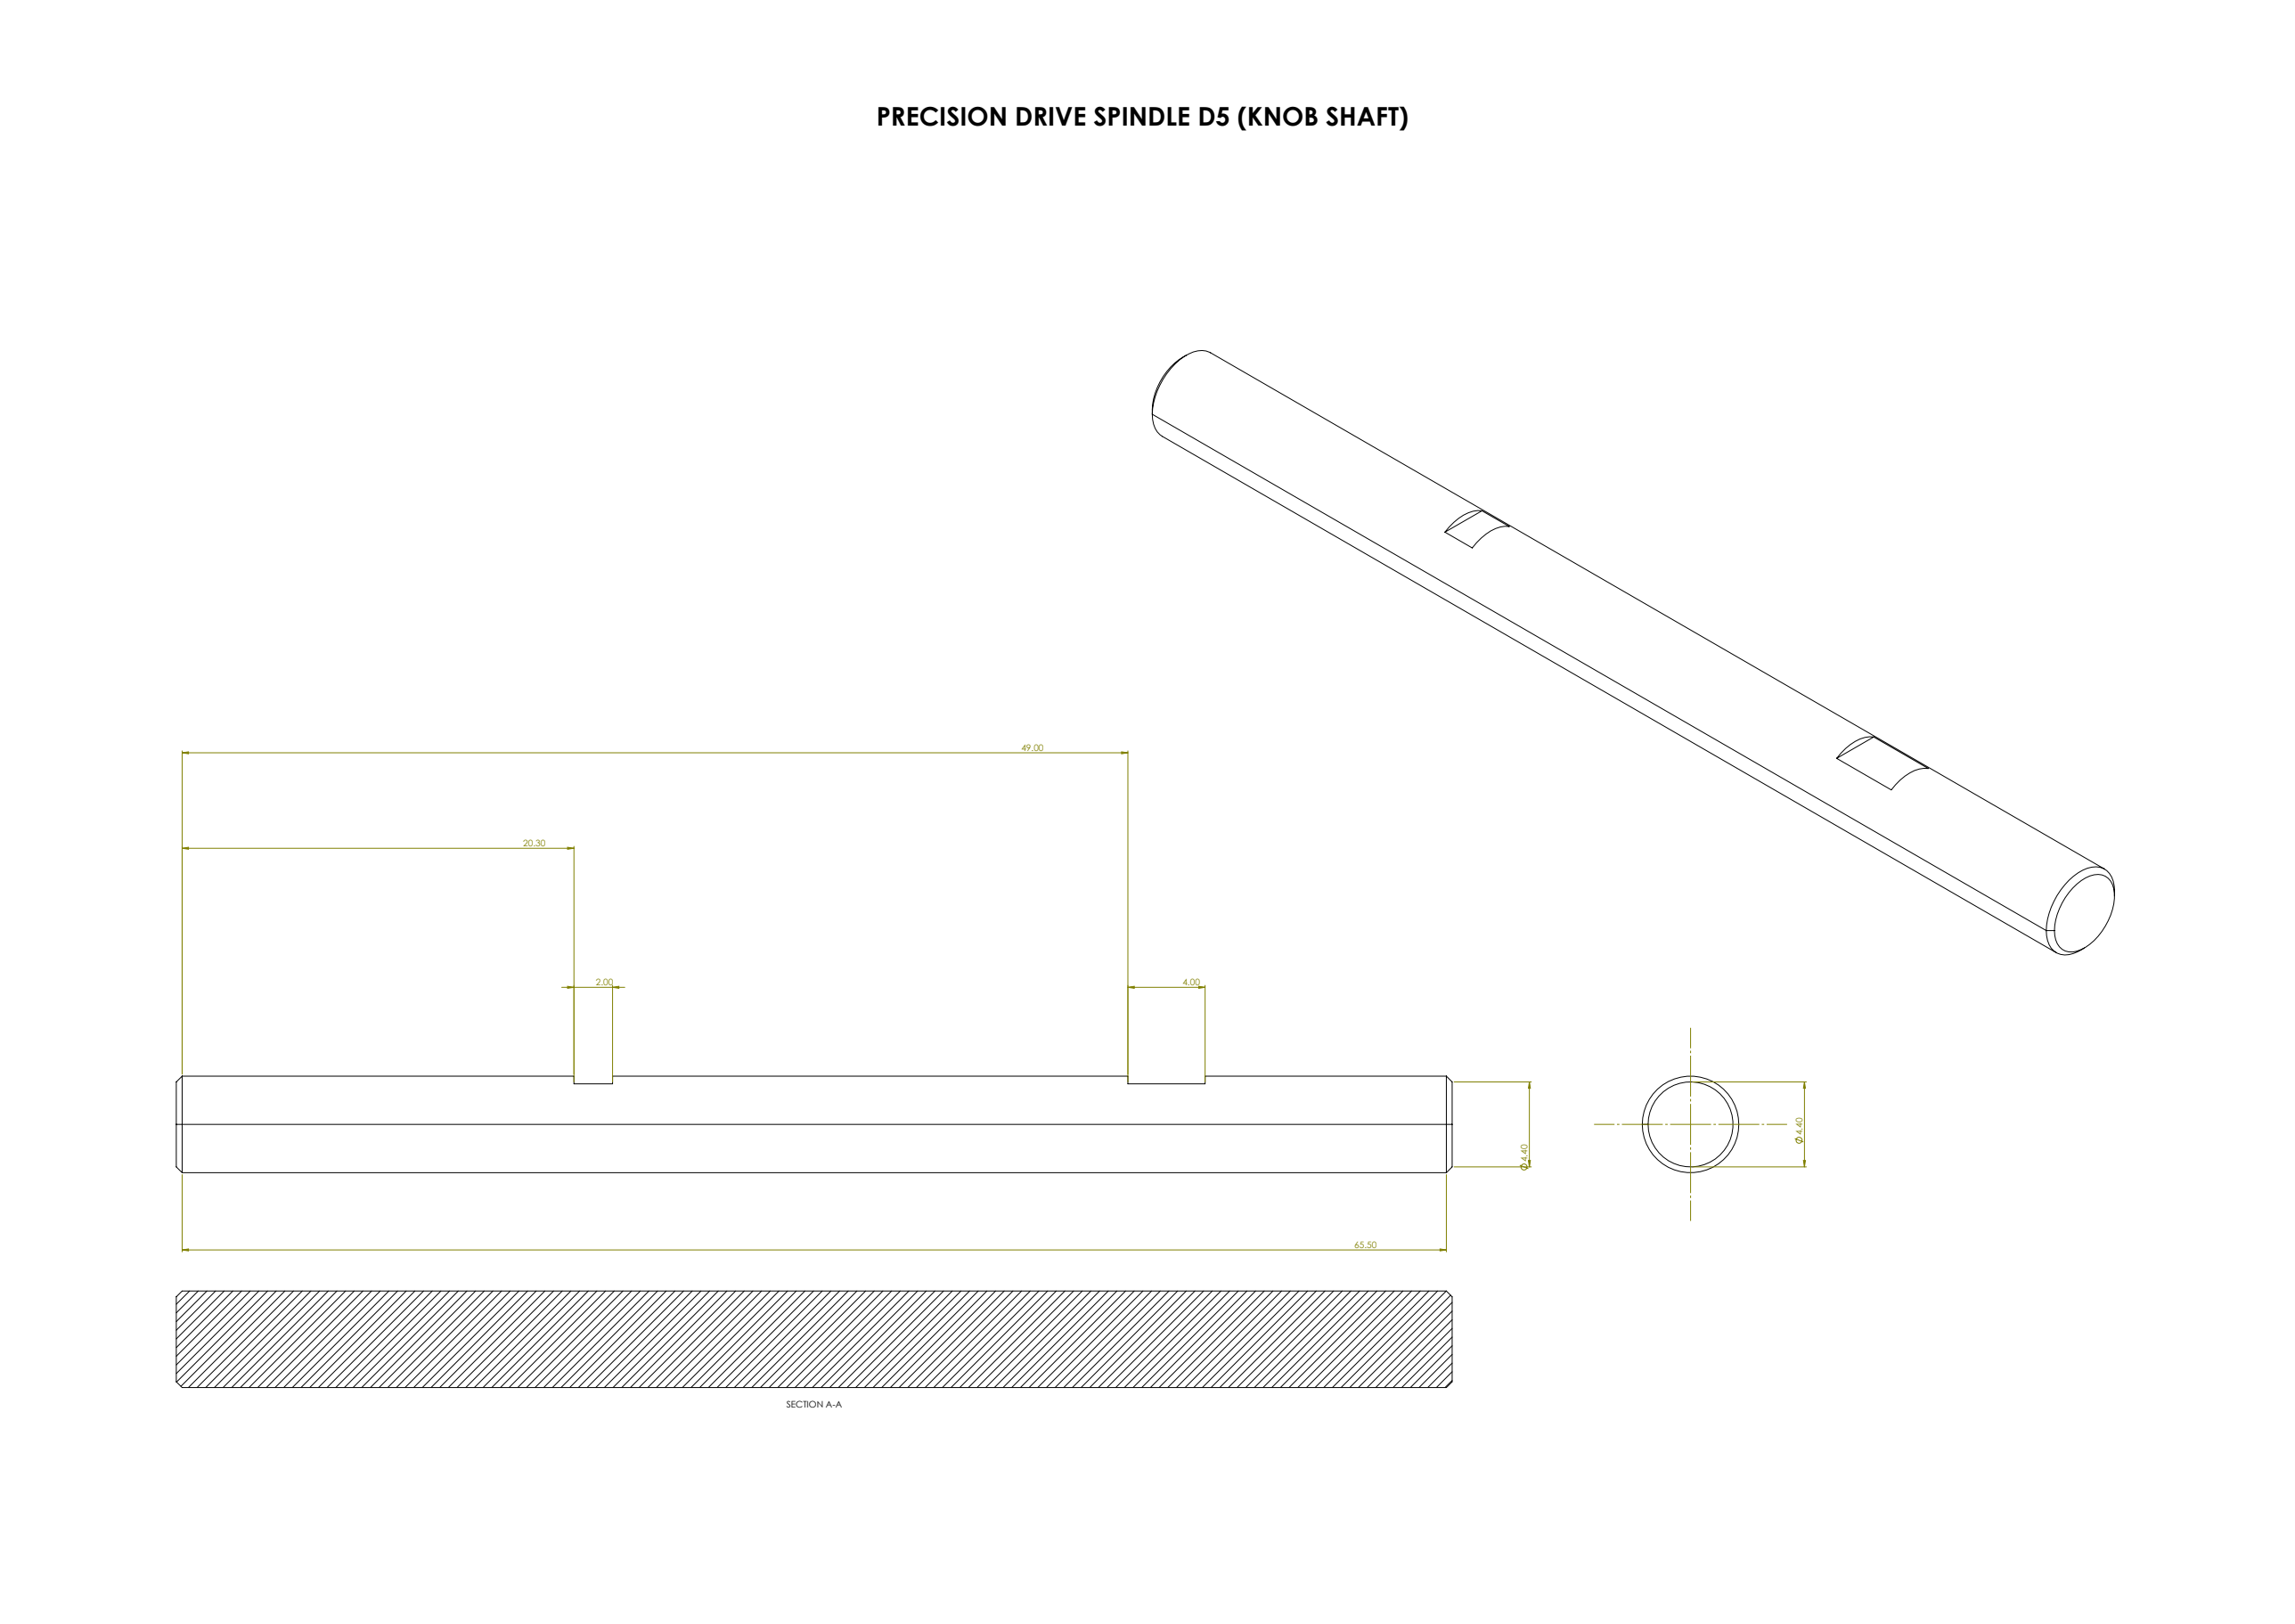
ISO-10303-21;
HEADER;
/* Generated by software containing ST-Developer
 * from STEP Tools, Inc. (www.steptools.com) 
 */

FILE_DESCRIPTION(
/* description */ (''),
/* implementation_level */ '2;1');

FILE_NAME(
/* name */ 'Precision Drive Spindle D5 (knob shaft).step',
/* time_stamp */ '2026-10-05T09:57:53+05:00',
/* author */ (''),
/* organization */ (''),
/* preprocessor_version */ 'ST-DEVELOPER v20.2',
/* originating_system */ 'Autodesk Translation Framework v15.15.0.0',
/* authorisation */ '');

FILE_SCHEMA (('AUTOMOTIVE_DESIGN { 1 0 10303 214 3 1 1 }'));
ENDSEC;

DATA;
#10=MECHANICAL_DESIGN_GEOMETRIC_PRESENTATION_REPRESENTATION('',(#554),#113984);
#518=SHAPE_REPRESENTATION_RELATIONSHIP('SRR','None',#114055,#536);
#536=ADVANCED_BREP_SHAPE_REPRESENTATION('',(#572),#113969);
#554=STYLED_ITEM('',(#114310),#572);
#572=MANIFOLD_SOLID_BREP('Precision Drive Spindle D5 (knob shaft)',#60395);
#635=CYLINDRICAL_SURFACE('',#61984,2.5);
#911=CONICAL_SURFACE('',#61982,2.34999999999999,0.785398163397437);
#912=CONICAL_SURFACE('',#61986,2.34999999999999,0.785398163397448);
#1055=CIRCLE('',#61971,2.5);
#1056=CIRCLE('',#61973,2.5);
#1057=CIRCLE('',#61976,2.5);
#1058=CIRCLE('',#61978,2.5);
#1059=CIRCLE('',#61981,2.20000000000001);
#1060=CIRCLE('',#61983,2.5);
#1061=CIRCLE('',#61985,2.5);
#1062=CIRCLE('',#61987,2.20000000000001);
#1825=FACE_BOUND('',#9526,.T.);
#1826=FACE_BOUND('',#9527,.T.);
#3035=PLANE('',#61970);
#3036=PLANE('',#61972);
#3037=PLANE('',#61974);
#3038=PLANE('',#61975);
#3039=PLANE('',#61977);
#3040=PLANE('',#61979);
#3041=PLANE('',#61980);
#3042=PLANE('',#61988);
#5967=FACE_OUTER_BOUND('',#9517,.T.);
#5968=FACE_OUTER_BOUND('',#9518,.T.);
#5969=FACE_OUTER_BOUND('',#9519,.T.);
#5970=FACE_OUTER_BOUND('',#9520,.T.);
#5971=FACE_OUTER_BOUND('',#9521,.T.);
#5972=FACE_OUTER_BOUND('',#9522,.T.);
#5973=FACE_OUTER_BOUND('',#9523,.T.);
#5974=FACE_OUTER_BOUND('',#9524,.T.);
#5975=FACE_OUTER_BOUND('',#9525,.T.);
#5976=FACE_OUTER_BOUND('',#9528,.T.);
#5977=FACE_OUTER_BOUND('',#9529,.T.);
#9517=EDGE_LOOP('',(#48949,#48950));
#9518=EDGE_LOOP('',(#48951,#48952));
#9519=EDGE_LOOP('',(#48953,#48954,#48955,#48956));
#9520=EDGE_LOOP('',(#48957,#48958));
#9521=EDGE_LOOP('',(#48959,#48960));
#9522=EDGE_LOOP('',(#48961,#48962,#48963,#48964));
#9523=EDGE_LOOP('',(#48965));
#9524=EDGE_LOOP('',(#48966,#48967,#48968,#48969));
#9525=EDGE_LOOP('',(#48970,#48971,#48972,#48973));
#9526=EDGE_LOOP('',(#48974,#48975,#48976,#48977));
#9527=EDGE_LOOP('',(#48978,#48979,#48980,#48981));
#9528=EDGE_LOOP('',(#48982,#48983,#48984,#48985));
#9529=EDGE_LOOP('',(#48986));
#14318=LINE('',#92618,#20352);
#14319=LINE('',#92623,#20353);
#14320=LINE('',#92625,#20354);
#14321=LINE('',#92626,#20355);
#14322=LINE('',#92631,#20356);
#14323=LINE('',#92636,#20357);
#14324=LINE('',#92638,#20358);
#14325=LINE('',#92639,#20359);
#14326=LINE('',#92646,#20360);
#14327=LINE('',#92650,#20361);
#14328=LINE('',#92654,#20362);
#20352=VECTOR('',#69944,10.);
#20353=VECTOR('',#69949,10.);
#20354=VECTOR('',#69952,10.);
#20355=VECTOR('',#69953,10.);
#20356=VECTOR('',#69958,10.);
#20357=VECTOR('',#69963,10.);
#20358=VECTOR('',#69966,10.);
#20359=VECTOR('',#69967,10.);
#20360=VECTOR('',#69976,2.34999999999999);
#20361=VECTOR('',#69981,2.5);
#20362=VECTOR('',#69986,2.34999999999999);
#27899=VERTEX_POINT('',#92615);
#27900=VERTEX_POINT('',#92616);
#27901=VERTEX_POINT('',#92620);
#27902=VERTEX_POINT('',#92621);
#27903=VERTEX_POINT('',#92628);
#27904=VERTEX_POINT('',#92629);
#27905=VERTEX_POINT('',#92633);
#27906=VERTEX_POINT('',#92634);
#27907=VERTEX_POINT('',#92641);
#27908=VERTEX_POINT('',#92644);
#27909=VERTEX_POINT('',#92648);
#27910=VERTEX_POINT('',#92652);
#35307=EDGE_CURVE('',#27899,#27900,#1055,.T.);
#35308=EDGE_CURVE('',#27899,#27900,#14318,.T.);
#35309=EDGE_CURVE('',#27901,#27902,#1056,.T.);
#35310=EDGE_CURVE('',#27901,#27902,#14319,.T.);
#35311=EDGE_CURVE('',#27902,#27899,#14320,.T.);
#35312=EDGE_CURVE('',#27900,#27901,#14321,.T.);
#35313=EDGE_CURVE('',#27903,#27904,#1057,.T.);
#35314=EDGE_CURVE('',#27903,#27904,#14322,.T.);
#35315=EDGE_CURVE('',#27905,#27906,#1058,.T.);
#35316=EDGE_CURVE('',#27905,#27906,#14323,.T.);
#35317=EDGE_CURVE('',#27906,#27903,#14324,.T.);
#35318=EDGE_CURVE('',#27904,#27905,#14325,.T.);
#35319=EDGE_CURVE('',#27907,#27907,#1059,.T.);
#35320=EDGE_CURVE('',#27908,#27908,#1060,.T.);
#35321=EDGE_CURVE('',#27908,#27907,#14326,.T.);
#35322=EDGE_CURVE('',#27909,#27909,#1061,.T.);
#35323=EDGE_CURVE('',#27909,#27908,#14327,.T.);
#35324=EDGE_CURVE('',#27910,#27910,#1062,.T.);
#35325=EDGE_CURVE('',#27910,#27909,#14328,.T.);
#48949=ORIENTED_EDGE('',*,*,#35307,.F.);
#48950=ORIENTED_EDGE('',*,*,#35308,.T.);
#48951=ORIENTED_EDGE('',*,*,#35309,.F.);
#48952=ORIENTED_EDGE('',*,*,#35310,.T.);
#48953=ORIENTED_EDGE('',*,*,#35311,.F.);
#48954=ORIENTED_EDGE('',*,*,#35310,.F.);
#48955=ORIENTED_EDGE('',*,*,#35312,.F.);
#48956=ORIENTED_EDGE('',*,*,#35308,.F.);
#48957=ORIENTED_EDGE('',*,*,#35313,.F.);
#48958=ORIENTED_EDGE('',*,*,#35314,.T.);
#48959=ORIENTED_EDGE('',*,*,#35315,.F.);
#48960=ORIENTED_EDGE('',*,*,#35316,.T.);
#48961=ORIENTED_EDGE('',*,*,#35317,.F.);
#48962=ORIENTED_EDGE('',*,*,#35316,.F.);
#48963=ORIENTED_EDGE('',*,*,#35318,.F.);
#48964=ORIENTED_EDGE('',*,*,#35314,.F.);
#48965=ORIENTED_EDGE('',*,*,#35319,.F.);
#48966=ORIENTED_EDGE('',*,*,#35320,.F.);
#48967=ORIENTED_EDGE('',*,*,#35321,.T.);
#48968=ORIENTED_EDGE('',*,*,#35319,.T.);
#48969=ORIENTED_EDGE('',*,*,#35321,.F.);
#48970=ORIENTED_EDGE('',*,*,#35322,.F.);
#48971=ORIENTED_EDGE('',*,*,#35323,.T.);
#48972=ORIENTED_EDGE('',*,*,#35320,.T.);
#48973=ORIENTED_EDGE('',*,*,#35323,.F.);
#48974=ORIENTED_EDGE('',*,*,#35309,.T.);
#48975=ORIENTED_EDGE('',*,*,#35311,.T.);
#48976=ORIENTED_EDGE('',*,*,#35307,.T.);
#48977=ORIENTED_EDGE('',*,*,#35312,.T.);
#48978=ORIENTED_EDGE('',*,*,#35315,.T.);
#48979=ORIENTED_EDGE('',*,*,#35317,.T.);
#48980=ORIENTED_EDGE('',*,*,#35313,.T.);
#48981=ORIENTED_EDGE('',*,*,#35318,.T.);
#48982=ORIENTED_EDGE('',*,*,#35324,.F.);
#48983=ORIENTED_EDGE('',*,*,#35325,.T.);
#48984=ORIENTED_EDGE('',*,*,#35322,.T.);
#48985=ORIENTED_EDGE('',*,*,#35325,.F.);
#48986=ORIENTED_EDGE('',*,*,#35324,.T.);
#59067=ADVANCED_FACE('',(#5967),#3035,.F.);
#59068=ADVANCED_FACE('',(#5968),#3036,.F.);
#59069=ADVANCED_FACE('',(#5969),#3037,.T.);
#59070=ADVANCED_FACE('',(#5970),#3038,.F.);
#59071=ADVANCED_FACE('',(#5971),#3039,.F.);
#59072=ADVANCED_FACE('',(#5972),#3040,.T.);
#59073=ADVANCED_FACE('',(#5973),#3041,.T.);
#59074=ADVANCED_FACE('',(#5974),#911,.T.);
#59075=ADVANCED_FACE('',(#5975,#1825,#1826),#635,.T.);
#59076=ADVANCED_FACE('',(#5976),#912,.T.);
#59077=ADVANCED_FACE('',(#5977),#3042,.T.);
#60395=CLOSED_SHELL('',(#59067,#59068,#59069,#59070,#59071,#59072,#59073,
#59074,#59075,#59076,#59077));
#61969=AXIS2_PLACEMENT_3D('',#92613,#69938,#69939);
#61970=AXIS2_PLACEMENT_3D('',#92614,#69940,#69941);
#61971=AXIS2_PLACEMENT_3D('',#92617,#69942,#69943);
#61972=AXIS2_PLACEMENT_3D('',#92619,#69945,#69946);
#61973=AXIS2_PLACEMENT_3D('',#92622,#69947,#69948);
#61974=AXIS2_PLACEMENT_3D('',#92624,#69950,#69951);
#61975=AXIS2_PLACEMENT_3D('',#92627,#69954,#69955);
#61976=AXIS2_PLACEMENT_3D('',#92630,#69956,#69957);
#61977=AXIS2_PLACEMENT_3D('',#92632,#69959,#69960);
#61978=AXIS2_PLACEMENT_3D('',#92635,#69961,#69962);
#61979=AXIS2_PLACEMENT_3D('',#92637,#69964,#69965);
#61980=AXIS2_PLACEMENT_3D('',#92640,#69968,#69969);
#61981=AXIS2_PLACEMENT_3D('',#92642,#69970,#69971);
#61982=AXIS2_PLACEMENT_3D('',#92643,#69972,#69973);
#61983=AXIS2_PLACEMENT_3D('',#92645,#69974,#69975);
#61984=AXIS2_PLACEMENT_3D('',#92647,#69977,#69978);
#61985=AXIS2_PLACEMENT_3D('',#92649,#69979,#69980);
#61986=AXIS2_PLACEMENT_3D('',#92651,#69982,#69983);
#61987=AXIS2_PLACEMENT_3D('',#92653,#69984,#69985);
#61988=AXIS2_PLACEMENT_3D('',#92655,#69987,#69988);
#69938=DIRECTION('axis',(0.,0.,1.));
#69939=DIRECTION('refdir',(1.,0.,0.));
#69940=DIRECTION('center_axis',(0.,0.,-1.));
#69941=DIRECTION('ref_axis',(-1.,0.,0.));
#69942=DIRECTION('center_axis',(0.,0.,-1.));
#69943=DIRECTION('ref_axis',(1.,0.,0.));
#69944=DIRECTION('',(1.,0.,0.));
#69945=DIRECTION('center_axis',(0.,0.,1.));
#69946=DIRECTION('ref_axis',(1.,0.,0.));
#69947=DIRECTION('center_axis',(0.,0.,1.));
#69948=DIRECTION('ref_axis',(1.,0.,0.));
#69949=DIRECTION('',(-1.,0.,0.));
#69950=DIRECTION('center_axis',(0.,1.,0.));
#69951=DIRECTION('ref_axis',(1.,0.,0.));
#69952=DIRECTION('',(0.,0.,-1.));
#69953=DIRECTION('',(0.,0.,1.));
#69954=DIRECTION('center_axis',(0.,0.,-1.));
#69955=DIRECTION('ref_axis',(-1.,0.,0.));
#69956=DIRECTION('center_axis',(0.,0.,-1.));
#69957=DIRECTION('ref_axis',(1.,0.,0.));
#69958=DIRECTION('',(1.,0.,0.));
#69959=DIRECTION('center_axis',(0.,0.,1.));
#69960=DIRECTION('ref_axis',(1.,0.,0.));
#69961=DIRECTION('center_axis',(0.,0.,1.));
#69962=DIRECTION('ref_axis',(1.,0.,0.));
#69963=DIRECTION('',(-1.,0.,0.));
#69964=DIRECTION('center_axis',(0.,1.,0.));
#69965=DIRECTION('ref_axis',(1.,0.,0.));
#69966=DIRECTION('',(0.,0.,-1.));
#69967=DIRECTION('',(0.,0.,1.));
#69968=DIRECTION('center_axis',(0.,0.,-1.));
#69969=DIRECTION('ref_axis',(-1.,0.,0.));
#69970=DIRECTION('center_axis',(0.,0.,1.));
#69971=DIRECTION('ref_axis',(1.,0.,0.));
#69972=DIRECTION('center_axis',(0.,0.,1.));
#69973=DIRECTION('ref_axis',(1.,0.,0.));
#69974=DIRECTION('center_axis',(0.,0.,1.));
#69975=DIRECTION('ref_axis',(1.,0.,0.));
#69976=DIRECTION('',(0.70710678118654,8.65956056235484E-17,-0.707106781186555));
#69977=DIRECTION('center_axis',(0.,0.,1.));
#69978=DIRECTION('ref_axis',(1.,0.,0.));
#69979=DIRECTION('center_axis',(0.,0.,1.));
#69980=DIRECTION('ref_axis',(1.,0.,0.));
#69981=DIRECTION('',(0.,0.,-1.));
#69982=DIRECTION('center_axis',(0.,0.,-1.));
#69983=DIRECTION('ref_axis',(1.,0.,0.));
#69984=DIRECTION('center_axis',(0.,0.,1.));
#69985=DIRECTION('ref_axis',(1.,0.,0.));
#69986=DIRECTION('',(-0.707106781186548,-8.65956056235493E-17,-0.707106781186548));
#69987=DIRECTION('center_axis',(0.,0.,1.));
#69988=DIRECTION('ref_axis',(1.,0.,0.));
#92613=CARTESIAN_POINT('',(0.,0.,0.));
#92614=CARTESIAN_POINT('Origin',(113.,20.1,61.));
#92615=CARTESIAN_POINT('',(108.643534003375,20.1,61.));
#92616=CARTESIAN_POINT('',(111.356465996625,20.1,61.));
#92617=CARTESIAN_POINT('Origin',(110.,18.,61.));
#92618=CARTESIAN_POINT('',(107.,20.1,61.));
#92619=CARTESIAN_POINT('Origin',(107.,20.1,65.));
#92620=CARTESIAN_POINT('',(111.356465996625,20.1,65.));
#92621=CARTESIAN_POINT('',(108.643534003375,20.1,65.));
#92622=CARTESIAN_POINT('Origin',(110.,18.,65.));
#92623=CARTESIAN_POINT('',(113.,20.1,65.));
#92624=CARTESIAN_POINT('Origin',(110.,20.1,63.));
#92625=CARTESIAN_POINT('',(108.643534003375,20.1,44.75));
#92626=CARTESIAN_POINT('',(111.356465996625,20.1,44.75));
#92627=CARTESIAN_POINT('Origin',(113.,20.1,32.3));
#92628=CARTESIAN_POINT('',(108.643534003375,20.1,32.3));
#92629=CARTESIAN_POINT('',(111.356465996625,20.1,32.3));
#92630=CARTESIAN_POINT('Origin',(110.,18.,32.3));
#92631=CARTESIAN_POINT('',(107.,20.1,32.3));
#92632=CARTESIAN_POINT('Origin',(107.,20.1,34.3));
#92633=CARTESIAN_POINT('',(111.356465996625,20.1,34.3));
#92634=CARTESIAN_POINT('',(108.643534003375,20.1,34.3));
#92635=CARTESIAN_POINT('Origin',(110.,18.,34.3));
#92636=CARTESIAN_POINT('',(113.,20.1,34.3));
#92637=CARTESIAN_POINT('Origin',(110.,20.1,33.3));
#92638=CARTESIAN_POINT('',(108.643534003375,20.1,44.75));
#92639=CARTESIAN_POINT('',(111.356465996625,20.1,44.75));
#92640=CARTESIAN_POINT('Origin',(112.2,18.,11.7));
#92641=CARTESIAN_POINT('',(107.8,18.,11.7));
#92642=CARTESIAN_POINT('Origin',(110.,18.,11.7));
#92643=CARTESIAN_POINT('Origin',(110.,18.,11.85));
#92644=CARTESIAN_POINT('',(107.5,18.,12.));
#92645=CARTESIAN_POINT('Origin',(110.,18.,12.));
#92646=CARTESIAN_POINT('',(107.65,18.,11.85));
#92647=CARTESIAN_POINT('Origin',(110.,18.,44.75));
#92648=CARTESIAN_POINT('',(107.5,18.,77.5));
#92649=CARTESIAN_POINT('Origin',(110.,18.,77.5));
#92650=CARTESIAN_POINT('',(107.5,18.,44.75));
#92651=CARTESIAN_POINT('Origin',(110.,18.,77.65));
#92652=CARTESIAN_POINT('',(107.8,18.,77.8));
#92653=CARTESIAN_POINT('Origin',(110.,18.,77.8));
#92654=CARTESIAN_POINT('',(107.65,18.,77.65));
#92655=CARTESIAN_POINT('Origin',(110.,18.,77.8));
#113949=UNCERTAINTY_MEASURE_WITH_UNIT(LENGTH_MEASURE(0.01),#113985,
'DISTANCE_ACCURACY_VALUE',
'Maximum model space distance between geometric entities at asserted c
onnectivities');
#113964=UNCERTAINTY_MEASURE_WITH_UNIT(LENGTH_MEASURE(0.01),#113985,
'DISTANCE_ACCURACY_VALUE',
'Maximum model space distance between geometric entities at asserted c
onnectivities');
#113969=(
GEOMETRIC_REPRESENTATION_CONTEXT(3)
GLOBAL_UNCERTAINTY_ASSIGNED_CONTEXT((#113949))
GLOBAL_UNIT_ASSIGNED_CONTEXT((#113985,#113987,#113988))
REPRESENTATION_CONTEXT('','3D')
);
#113984=(
GEOMETRIC_REPRESENTATION_CONTEXT(3)
GLOBAL_UNCERTAINTY_ASSIGNED_CONTEXT((#113964))
GLOBAL_UNIT_ASSIGNED_CONTEXT((#113985,#113987,#113988))
REPRESENTATION_CONTEXT('','3D')
);
#113985=(
LENGTH_UNIT()
NAMED_UNIT(*)
SI_UNIT(.MILLI.,.METRE.)
);
#113987=(
NAMED_UNIT(*)
PLANE_ANGLE_UNIT()
SI_UNIT($,.RADIAN.)
);
#113988=(
NAMED_UNIT(*)
SI_UNIT($,.STERADIAN.)
SOLID_ANGLE_UNIT()
);
#113993=SHAPE_DEFINITION_REPRESENTATION(#114012,#114055);
#114012=PRODUCT_DEFINITION_SHAPE('',$,#114075);
#114055=SHAPE_REPRESENTATION('',(#61969),#113969);
#114070=PRODUCT_DEFINITION_CONTEXT('part definition',#114129,'design');
#114075=PRODUCT_DEFINITION('2026-10-05-09-49-04-660',
'Precision Drive Spindle D5 (knob shaft)',#114094,#114070);
#114094=PRODUCT_DEFINITION_FORMATION('',$,#114135);
#114129=APPLICATION_CONTEXT(
'Core Data for Automotive Mechanical Design Process');
#114130=PRODUCT_CONTEXT('part definition',#114129,'mechanical');
#114135=PRODUCT('2026-10-05-09-49-04-660',
'Precision Drive Spindle D5 (knob shaft)',$,(#114130));
#114304=COLOUR_RGB('Grey',0.48,0.52,0.57);
#114305=FILL_AREA_STYLE_COLOUR('',#114304);
#114306=FILL_AREA_STYLE('',(#114305));
#114307=SURFACE_STYLE_FILL_AREA(#114306);
#114308=SURFACE_SIDE_STYLE('',(#114307));
#114309=SURFACE_STYLE_USAGE(.BOTH.,#114308);
#114310=PRESENTATION_STYLE_ASSIGNMENT((#114309));
ENDSEC;
END-ISO-10303-21;
